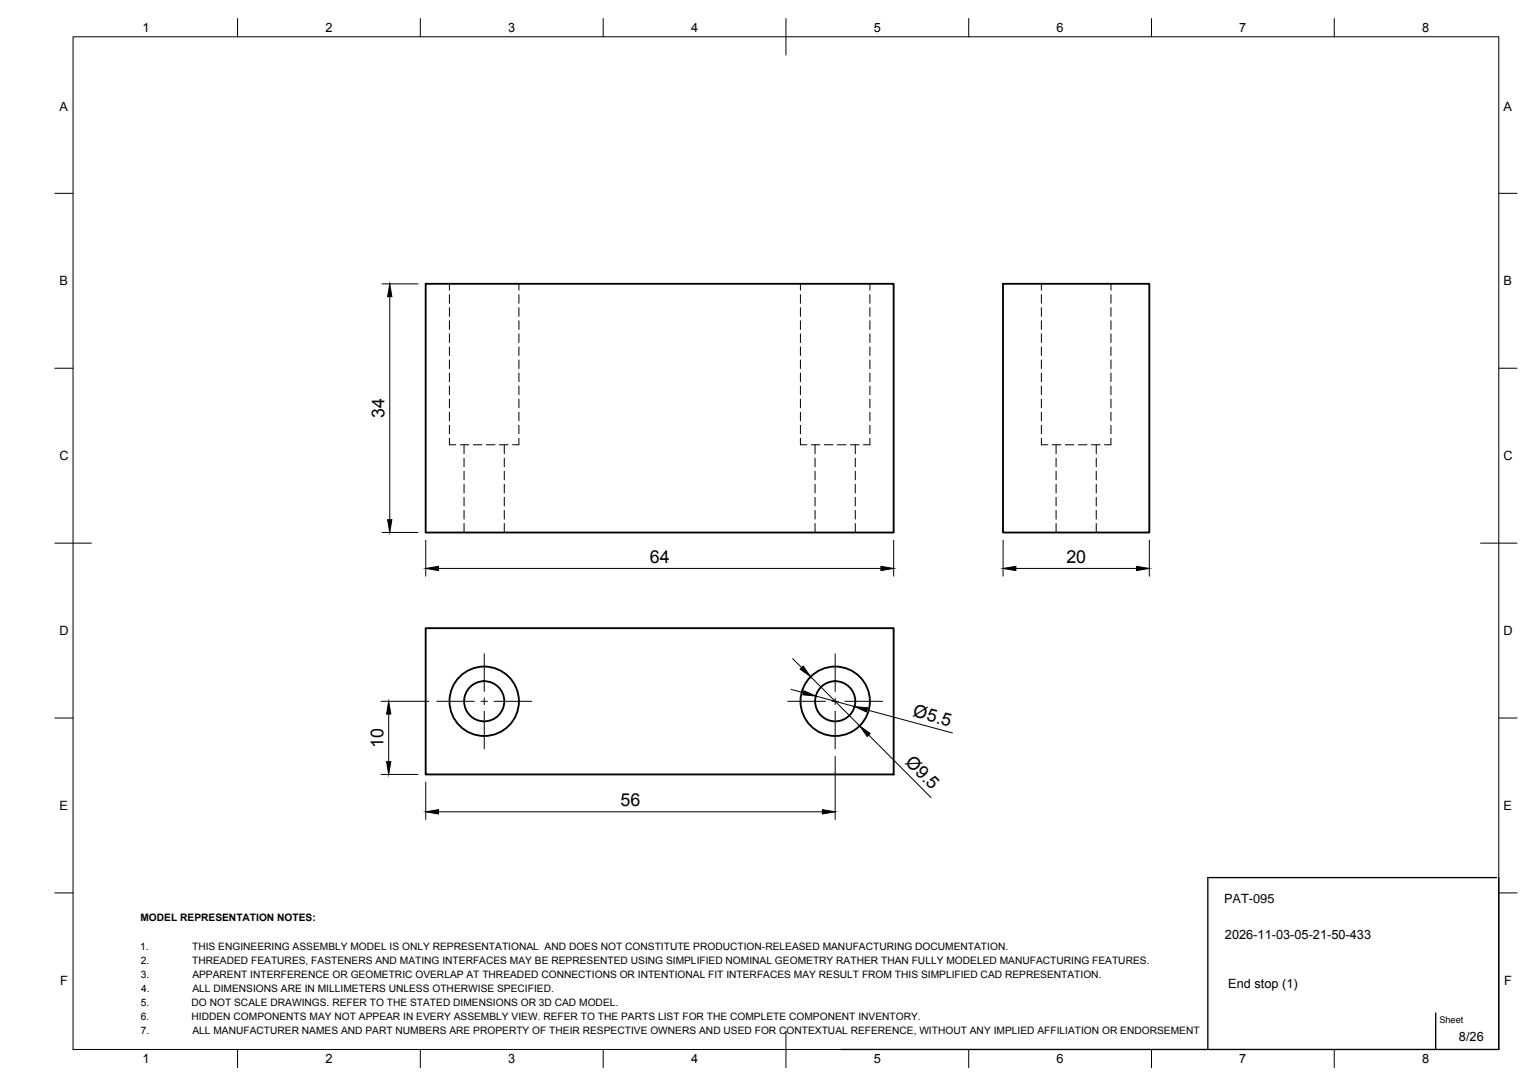
ISO-10303-21;
HEADER;
/* Generated by software containing ST-Developer
 * from STEP Tools, Inc. (www.steptools.com) 
 */

FILE_DESCRIPTION(
/* description */ ('Single-Axis Profile-Rail Linear Slide'),
/* implementation_level */ '2;1');

FILE_NAME(
/* name */ 'End stop (1).step',
/* time_stamp */ '2026-10-27T10:47:43-07:00',
/* author */ (''),
/* organization */ (''),
/* preprocessor_version */ 'ST-DEVELOPER v20.2',
/* originating_system */ 'Autodesk Translation Framework v15.17.0.0',
/* authorisation */ '');

FILE_SCHEMA (('AUTOMOTIVE_DESIGN { 1 0 10303 214 3 1 1 }'));
ENDSEC;

DATA;
#10=MECHANICAL_DESIGN_GEOMETRIC_PRESENTATION_REPRESENTATION('',(#332),#14478);
#278=SHAPE_REPRESENTATION_RELATIONSHIP('SRR','None',#14608,#305);
#305=ADVANCED_BREP_SHAPE_REPRESENTATION('',(#359),#14452);
#332=STYLED_ITEM('',(#14824),#359);
#359=MANIFOLD_SOLID_BREP('Body1',#8592);
#412=FACE_BOUND('',#1369,.T.);
#413=FACE_BOUND('',#1372,.T.);
#414=FACE_BOUND('',#1380,.T.);
#415=FACE_BOUND('',#1381,.T.);
#416=FACE_BOUND('',#1383,.T.);
#417=FACE_BOUND('',#1384,.T.);
#488=PLANE('',#9002);
#489=PLANE('',#9007);
#490=PLANE('',#9013);
#491=PLANE('',#9014);
#492=PLANE('',#9015);
#493=PLANE('',#9016);
#494=PLANE('',#9017);
#495=PLANE('',#9018);
#878=FACE_OUTER_BOUND('',#1367,.T.);
#879=FACE_OUTER_BOUND('',#1368,.T.);
#880=FACE_OUTER_BOUND('',#1370,.T.);
#881=FACE_OUTER_BOUND('',#1371,.T.);
#882=FACE_OUTER_BOUND('',#1373,.T.);
#883=FACE_OUTER_BOUND('',#1374,.T.);
#884=FACE_OUTER_BOUND('',#1375,.T.);
#885=FACE_OUTER_BOUND('',#1376,.T.);
#886=FACE_OUTER_BOUND('',#1377,.T.);
#887=FACE_OUTER_BOUND('',#1378,.T.);
#888=FACE_OUTER_BOUND('',#1379,.T.);
#889=FACE_OUTER_BOUND('',#1382,.T.);
#1367=EDGE_LOOP('',(#5993,#5994,#5995,#5996));
#1368=EDGE_LOOP('',(#5997));
#1369=EDGE_LOOP('',(#5998));
#1370=EDGE_LOOP('',(#5999,#6000,#6001,#6002));
#1371=EDGE_LOOP('',(#6003));
#1372=EDGE_LOOP('',(#6004));
#1373=EDGE_LOOP('',(#6005,#6006,#6007,#6008));
#1374=EDGE_LOOP('',(#6009,#6010,#6011,#6012));
#1375=EDGE_LOOP('',(#6013,#6014,#6015,#6016));
#1376=EDGE_LOOP('',(#6017,#6018,#6019,#6020));
#1377=EDGE_LOOP('',(#6021,#6022,#6023,#6024));
#1378=EDGE_LOOP('',(#6025,#6026,#6027,#6028));
#1379=EDGE_LOOP('',(#6029,#6030,#6031,#6032));
#1380=EDGE_LOOP('',(#6033));
#1381=EDGE_LOOP('',(#6034));
#1382=EDGE_LOOP('',(#6035,#6036,#6037,#6038));
#1383=EDGE_LOOP('',(#6039));
#1384=EDGE_LOOP('',(#6040));
#1894=LINE('',#12194,#2865);
#1895=LINE('',#12203,#2866);
#1896=LINE('',#12211,#2867);
#1897=LINE('',#12215,#2868);
#1898=LINE('',#12219,#2869);
#1899=LINE('',#12221,#2870);
#1900=LINE('',#12223,#2871);
#1901=LINE('',#12224,#2872);
#1902=LINE('',#12227,#2873);
#1903=LINE('',#12229,#2874);
#1904=LINE('',#12230,#2875);
#1905=LINE('',#12233,#2876);
#1906=LINE('',#12235,#2877);
#1907=LINE('',#12236,#2878);
#1908=LINE('',#12238,#2879);
#1909=LINE('',#12239,#2880);
#2865=VECTOR('',#9839,0.475000000000001);
#2866=VECTOR('',#9850,0.475000000000001);
#2867=VECTOR('',#9861,0.274999999999999);
#2868=VECTOR('',#9866,0.274999999999999);
#2869=VECTOR('',#9869,1.);
#2870=VECTOR('',#9870,1.);
#2871=VECTOR('',#9871,1.);
#2872=VECTOR('',#9872,1.);
#2873=VECTOR('',#9875,1.);
#2874=VECTOR('',#9876,1.);
#2875=VECTOR('',#9877,1.);
#2876=VECTOR('',#9880,1.);
#2877=VECTOR('',#9881,1.);
#2878=VECTOR('',#9882,1.);
#2879=VECTOR('',#9885,1.);
#2880=VECTOR('',#9886,1.);
#3818=CIRCLE('',#9000,0.475000000000001);
#3819=CIRCLE('',#9001,0.475000000000001);
#3820=CIRCLE('',#9003,0.274999999999999);
#3821=CIRCLE('',#9005,0.475000000000001);
#3822=CIRCLE('',#9006,0.475000000000001);
#3823=CIRCLE('',#9008,0.274999999999999);
#3824=CIRCLE('',#9010,0.274999999999999);
#3825=CIRCLE('',#9012,0.274999999999999);
#3998=VERTEX_POINT('',#12191);
#3999=VERTEX_POINT('',#12193);
#4000=VERTEX_POINT('',#12197);
#4001=VERTEX_POINT('',#12200);
#4002=VERTEX_POINT('',#12202);
#4003=VERTEX_POINT('',#12206);
#4004=VERTEX_POINT('',#12209);
#4005=VERTEX_POINT('',#12213);
#4006=VERTEX_POINT('',#12217);
#4007=VERTEX_POINT('',#12218);
#4008=VERTEX_POINT('',#12220);
#4009=VERTEX_POINT('',#12222);
#4010=VERTEX_POINT('',#12226);
#4011=VERTEX_POINT('',#12228);
#4012=VERTEX_POINT('',#12232);
#4013=VERTEX_POINT('',#12234);
#4774=EDGE_CURVE('',#3998,#3998,#3818,.T.);
#4775=EDGE_CURVE('',#3998,#3999,#1894,.T.);
#4776=EDGE_CURVE('',#3999,#3999,#3819,.T.);
#4777=EDGE_CURVE('',#4000,#4000,#3820,.T.);
#4778=EDGE_CURVE('',#4001,#4001,#3821,.T.);
#4779=EDGE_CURVE('',#4001,#4002,#1895,.T.);
#4780=EDGE_CURVE('',#4002,#4002,#3822,.T.);
#4781=EDGE_CURVE('',#4003,#4003,#3823,.T.);
#4782=EDGE_CURVE('',#4004,#4004,#3824,.T.);
#4783=EDGE_CURVE('',#4004,#4000,#1896,.T.);
#4784=EDGE_CURVE('',#4005,#4005,#3825,.T.);
#4785=EDGE_CURVE('',#4005,#4003,#1897,.T.);
#4786=EDGE_CURVE('',#4006,#4007,#1898,.T.);
#4787=EDGE_CURVE('',#4007,#4008,#1899,.T.);
#4788=EDGE_CURVE('',#4009,#4008,#1900,.T.);
#4789=EDGE_CURVE('',#4006,#4009,#1901,.T.);
#4790=EDGE_CURVE('',#4010,#4006,#1902,.T.);
#4791=EDGE_CURVE('',#4011,#4009,#1903,.T.);
#4792=EDGE_CURVE('',#4010,#4011,#1904,.T.);
#4793=EDGE_CURVE('',#4012,#4010,#1905,.T.);
#4794=EDGE_CURVE('',#4013,#4011,#1906,.T.);
#4795=EDGE_CURVE('',#4012,#4013,#1907,.T.);
#4796=EDGE_CURVE('',#4007,#4012,#1908,.T.);
#4797=EDGE_CURVE('',#4008,#4013,#1909,.T.);
#5993=ORIENTED_EDGE('',*,*,#4774,.F.);
#5994=ORIENTED_EDGE('',*,*,#4775,.T.);
#5995=ORIENTED_EDGE('',*,*,#4776,.F.);
#5996=ORIENTED_EDGE('',*,*,#4775,.F.);
#5997=ORIENTED_EDGE('',*,*,#4774,.T.);
#5998=ORIENTED_EDGE('',*,*,#4777,.F.);
#5999=ORIENTED_EDGE('',*,*,#4778,.F.);
#6000=ORIENTED_EDGE('',*,*,#4779,.T.);
#6001=ORIENTED_EDGE('',*,*,#4780,.F.);
#6002=ORIENTED_EDGE('',*,*,#4779,.F.);
#6003=ORIENTED_EDGE('',*,*,#4778,.T.);
#6004=ORIENTED_EDGE('',*,*,#4781,.F.);
#6005=ORIENTED_EDGE('',*,*,#4782,.F.);
#6006=ORIENTED_EDGE('',*,*,#4783,.T.);
#6007=ORIENTED_EDGE('',*,*,#4777,.T.);
#6008=ORIENTED_EDGE('',*,*,#4783,.F.);
#6009=ORIENTED_EDGE('',*,*,#4784,.F.);
#6010=ORIENTED_EDGE('',*,*,#4785,.T.);
#6011=ORIENTED_EDGE('',*,*,#4781,.T.);
#6012=ORIENTED_EDGE('',*,*,#4785,.F.);
#6013=ORIENTED_EDGE('',*,*,#4786,.T.);
#6014=ORIENTED_EDGE('',*,*,#4787,.T.);
#6015=ORIENTED_EDGE('',*,*,#4788,.F.);
#6016=ORIENTED_EDGE('',*,*,#4789,.F.);
#6017=ORIENTED_EDGE('',*,*,#4790,.T.);
#6018=ORIENTED_EDGE('',*,*,#4789,.T.);
#6019=ORIENTED_EDGE('',*,*,#4791,.F.);
#6020=ORIENTED_EDGE('',*,*,#4792,.F.);
#6021=ORIENTED_EDGE('',*,*,#4793,.T.);
#6022=ORIENTED_EDGE('',*,*,#4792,.T.);
#6023=ORIENTED_EDGE('',*,*,#4794,.F.);
#6024=ORIENTED_EDGE('',*,*,#4795,.F.);
#6025=ORIENTED_EDGE('',*,*,#4796,.T.);
#6026=ORIENTED_EDGE('',*,*,#4795,.T.);
#6027=ORIENTED_EDGE('',*,*,#4797,.F.);
#6028=ORIENTED_EDGE('',*,*,#4787,.F.);
#6029=ORIENTED_EDGE('',*,*,#4797,.T.);
#6030=ORIENTED_EDGE('',*,*,#4794,.T.);
#6031=ORIENTED_EDGE('',*,*,#4791,.T.);
#6032=ORIENTED_EDGE('',*,*,#4788,.T.);
#6033=ORIENTED_EDGE('',*,*,#4776,.T.);
#6034=ORIENTED_EDGE('',*,*,#4780,.T.);
#6035=ORIENTED_EDGE('',*,*,#4796,.F.);
#6036=ORIENTED_EDGE('',*,*,#4786,.F.);
#6037=ORIENTED_EDGE('',*,*,#4790,.F.);
#6038=ORIENTED_EDGE('',*,*,#4793,.F.);
#6039=ORIENTED_EDGE('',*,*,#4782,.T.);
#6040=ORIENTED_EDGE('',*,*,#4784,.T.);
#8089=CYLINDRICAL_SURFACE('',#8999,0.475000000000001);
#8090=CYLINDRICAL_SURFACE('',#9004,0.475000000000001);
#8091=CYLINDRICAL_SURFACE('',#9009,0.274999999999999);
#8092=CYLINDRICAL_SURFACE('',#9011,0.274999999999999);
#8172=ADVANCED_FACE('',(#878),#8089,.F.);
#8173=ADVANCED_FACE('',(#879,#412),#488,.T.);
#8174=ADVANCED_FACE('',(#880),#8090,.F.);
#8175=ADVANCED_FACE('',(#881,#413),#489,.T.);
#8176=ADVANCED_FACE('',(#882),#8091,.F.);
#8177=ADVANCED_FACE('',(#883),#8092,.F.);
#8178=ADVANCED_FACE('',(#884),#490,.T.);
#8179=ADVANCED_FACE('',(#885),#491,.T.);
#8180=ADVANCED_FACE('',(#886),#492,.T.);
#8181=ADVANCED_FACE('',(#887),#493,.T.);
#8182=ADVANCED_FACE('',(#888,#414,#415),#494,.T.);
#8183=ADVANCED_FACE('',(#889,#416,#417),#495,.F.);
#8592=CLOSED_SHELL('',(#8172,#8173,#8174,#8175,#8176,#8177,#8178,#8179,
#8180,#8181,#8182,#8183));
#8998=AXIS2_PLACEMENT_3D('',#12189,#9833,#9834);
#8999=AXIS2_PLACEMENT_3D('',#12190,#9835,#9836);
#9000=AXIS2_PLACEMENT_3D('',#12192,#9837,#9838);
#9001=AXIS2_PLACEMENT_3D('',#12195,#9840,#9841);
#9002=AXIS2_PLACEMENT_3D('',#12196,#9842,#9843);
#9003=AXIS2_PLACEMENT_3D('',#12198,#9844,#9845);
#9004=AXIS2_PLACEMENT_3D('',#12199,#9846,#9847);
#9005=AXIS2_PLACEMENT_3D('',#12201,#9848,#9849);
#9006=AXIS2_PLACEMENT_3D('',#12204,#9851,#9852);
#9007=AXIS2_PLACEMENT_3D('',#12205,#9853,#9854);
#9008=AXIS2_PLACEMENT_3D('',#12207,#9855,#9856);
#9009=AXIS2_PLACEMENT_3D('',#12208,#9857,#9858);
#9010=AXIS2_PLACEMENT_3D('',#12210,#9859,#9860);
#9011=AXIS2_PLACEMENT_3D('',#12212,#9862,#9863);
#9012=AXIS2_PLACEMENT_3D('',#12214,#9864,#9865);
#9013=AXIS2_PLACEMENT_3D('',#12216,#9867,#9868);
#9014=AXIS2_PLACEMENT_3D('',#12225,#9873,#9874);
#9015=AXIS2_PLACEMENT_3D('',#12231,#9878,#9879);
#9016=AXIS2_PLACEMENT_3D('',#12237,#9883,#9884);
#9017=AXIS2_PLACEMENT_3D('',#12240,#9887,#9888);
#9018=AXIS2_PLACEMENT_3D('',#12241,#9889,#9890);
#9833=DIRECTION('axis',(0.,0.,1.));
#9834=DIRECTION('refdir',(1.,0.,0.));
#9835=DIRECTION('center_axis',(0.,0.,1.));
#9836=DIRECTION('ref_axis',(1.,0.,0.));
#9837=DIRECTION('center_axis',(0.,0.,1.));
#9838=DIRECTION('ref_axis',(1.,0.,0.));
#9839=DIRECTION('',(0.,0.,1.));
#9840=DIRECTION('center_axis',(0.,0.,-1.));
#9841=DIRECTION('ref_axis',(1.,0.,0.));
#9842=DIRECTION('center_axis',(0.,0.,1.));
#9843=DIRECTION('ref_axis',(1.,0.,0.));
#9844=DIRECTION('center_axis',(0.,0.,1.));
#9845=DIRECTION('ref_axis',(1.,0.,0.));
#9846=DIRECTION('center_axis',(0.,0.,1.));
#9847=DIRECTION('ref_axis',(1.,0.,0.));
#9848=DIRECTION('center_axis',(0.,0.,1.));
#9849=DIRECTION('ref_axis',(1.,0.,0.));
#9850=DIRECTION('',(0.,0.,1.));
#9851=DIRECTION('center_axis',(0.,0.,-1.));
#9852=DIRECTION('ref_axis',(1.,0.,0.));
#9853=DIRECTION('center_axis',(0.,0.,1.));
#9854=DIRECTION('ref_axis',(1.,0.,0.));
#9855=DIRECTION('center_axis',(0.,0.,1.));
#9856=DIRECTION('ref_axis',(1.,0.,0.));
#9857=DIRECTION('center_axis',(0.,0.,1.));
#9858=DIRECTION('ref_axis',(1.,0.,0.));
#9859=DIRECTION('center_axis',(0.,0.,1.));
#9860=DIRECTION('ref_axis',(1.,0.,0.));
#9861=DIRECTION('',(0.,0.,1.));
#9862=DIRECTION('center_axis',(0.,0.,1.));
#9863=DIRECTION('ref_axis',(1.,0.,0.));
#9864=DIRECTION('center_axis',(0.,0.,1.));
#9865=DIRECTION('ref_axis',(1.,0.,0.));
#9866=DIRECTION('',(0.,0.,1.));
#9867=DIRECTION('center_axis',(0.,1.,0.));
#9868=DIRECTION('ref_axis',(-1.,0.,0.));
#9869=DIRECTION('',(-1.,0.,0.));
#9870=DIRECTION('',(0.,0.,1.));
#9871=DIRECTION('',(-1.,0.,0.));
#9872=DIRECTION('',(0.,0.,1.));
#9873=DIRECTION('center_axis',(1.,0.,0.));
#9874=DIRECTION('ref_axis',(0.,1.,0.));
#9875=DIRECTION('',(0.,1.,0.));
#9876=DIRECTION('',(0.,1.,0.));
#9877=DIRECTION('',(0.,0.,1.));
#9878=DIRECTION('center_axis',(0.,-1.,0.));
#9879=DIRECTION('ref_axis',(1.,0.,0.));
#9880=DIRECTION('',(1.,0.,0.));
#9881=DIRECTION('',(1.,0.,0.));
#9882=DIRECTION('',(0.,0.,1.));
#9883=DIRECTION('center_axis',(-1.,0.,0.));
#9884=DIRECTION('ref_axis',(0.,-1.,0.));
#9885=DIRECTION('',(0.,-1.,0.));
#9886=DIRECTION('',(0.,-1.,0.));
#9887=DIRECTION('center_axis',(0.,0.,1.));
#9888=DIRECTION('ref_axis',(1.,0.,0.));
#9889=DIRECTION('center_axis',(0.,0.,1.));
#9890=DIRECTION('ref_axis',(1.,0.,0.));
#12189=CARTESIAN_POINT('',(0.,0.,0.));
#12190=CARTESIAN_POINT('Origin',(23.,-2.4,4.));
#12191=CARTESIAN_POINT('',(22.525,-2.4,4.));
#12192=CARTESIAN_POINT('Origin',(23.,-2.4,4.));
#12193=CARTESIAN_POINT('',(22.525,-2.4,6.2));
#12194=CARTESIAN_POINT('',(22.525,-2.4,4.));
#12195=CARTESIAN_POINT('Origin',(23.,-2.4,6.2));
#12196=CARTESIAN_POINT('Origin',(23.,-2.4,4.));
#12197=CARTESIAN_POINT('',(22.725,-2.4,4.));
#12198=CARTESIAN_POINT('Origin',(23.,-2.4,4.));
#12199=CARTESIAN_POINT('Origin',(23.,2.4,4.));
#12200=CARTESIAN_POINT('',(22.525,2.4,4.));
#12201=CARTESIAN_POINT('Origin',(23.,2.4,4.));
#12202=CARTESIAN_POINT('',(22.525,2.4,6.2));
#12203=CARTESIAN_POINT('',(22.525,2.4,4.));
#12204=CARTESIAN_POINT('Origin',(23.,2.4,6.2));
#12205=CARTESIAN_POINT('Origin',(23.,2.4,4.));
#12206=CARTESIAN_POINT('',(22.725,2.4,4.));
#12207=CARTESIAN_POINT('Origin',(23.,2.4,4.));
#12208=CARTESIAN_POINT('Origin',(23.,-2.4,2.7));
#12209=CARTESIAN_POINT('',(22.725,-2.4,2.8));
#12210=CARTESIAN_POINT('Origin',(23.,-2.4,2.8));
#12211=CARTESIAN_POINT('',(22.725,-2.4,2.7));
#12212=CARTESIAN_POINT('Origin',(23.,2.4,2.7));
#12213=CARTESIAN_POINT('',(22.725,2.4,2.8));
#12214=CARTESIAN_POINT('Origin',(23.,2.4,2.8));
#12215=CARTESIAN_POINT('',(22.725,2.4,2.7));
#12216=CARTESIAN_POINT('Origin',(24.,3.2,2.8));
#12217=CARTESIAN_POINT('',(24.,3.2,2.8));
#12218=CARTESIAN_POINT('',(22.,3.2,2.8));
#12219=CARTESIAN_POINT('',(24.,3.2,2.8));
#12220=CARTESIAN_POINT('',(22.,3.2,6.2));
#12221=CARTESIAN_POINT('',(22.,3.2,2.8));
#12222=CARTESIAN_POINT('',(24.,3.2,6.2));
#12223=CARTESIAN_POINT('',(24.,3.2,6.2));
#12224=CARTESIAN_POINT('',(24.,3.2,2.8));
#12225=CARTESIAN_POINT('Origin',(24.,-3.2,2.8));
#12226=CARTESIAN_POINT('',(24.,-3.2,2.8));
#12227=CARTESIAN_POINT('',(24.,-3.2,2.8));
#12228=CARTESIAN_POINT('',(24.,-3.2,6.2));
#12229=CARTESIAN_POINT('',(24.,-3.2,6.2));
#12230=CARTESIAN_POINT('',(24.,-3.2,2.8));
#12231=CARTESIAN_POINT('Origin',(22.,-3.2,2.8));
#12232=CARTESIAN_POINT('',(22.,-3.2,2.8));
#12233=CARTESIAN_POINT('',(22.,-3.2,2.8));
#12234=CARTESIAN_POINT('',(22.,-3.2,6.2));
#12235=CARTESIAN_POINT('',(22.,-3.2,6.2));
#12236=CARTESIAN_POINT('',(22.,-3.2,2.8));
#12237=CARTESIAN_POINT('Origin',(22.,3.2,2.8));
#12238=CARTESIAN_POINT('',(22.,3.2,2.8));
#12239=CARTESIAN_POINT('',(22.,3.2,6.2));
#12240=CARTESIAN_POINT('Origin',(23.,0.,6.2));
#12241=CARTESIAN_POINT('Origin',(23.,0.,2.8));
#14420=UNCERTAINTY_MEASURE_WITH_UNIT(LENGTH_MEASURE(0.001),#14479,
'DISTANCE_ACCURACY_VALUE',
'Maximum model space distance between geometric entities at asserted c
onnectivities');
#14446=UNCERTAINTY_MEASURE_WITH_UNIT(LENGTH_MEASURE(0.001),#14479,
'DISTANCE_ACCURACY_VALUE',
'Maximum model space distance between geometric entities at asserted c
onnectivities');
#14452=(
GEOMETRIC_REPRESENTATION_CONTEXT(3)
GLOBAL_UNCERTAINTY_ASSIGNED_CONTEXT((#14420))
GLOBAL_UNIT_ASSIGNED_CONTEXT((#14479,#14481,#14482))
REPRESENTATION_CONTEXT('','3D')
);
#14478=(
GEOMETRIC_REPRESENTATION_CONTEXT(3)
GLOBAL_UNCERTAINTY_ASSIGNED_CONTEXT((#14446))
GLOBAL_UNIT_ASSIGNED_CONTEXT((#14479,#14481,#14482))
REPRESENTATION_CONTEXT('','3D')
);
#14479=(
LENGTH_UNIT()
NAMED_UNIT(*)
SI_UNIT(.CENTI.,.METRE.)
);
#14481=(
NAMED_UNIT(*)
PLANE_ANGLE_UNIT()
SI_UNIT($,.RADIAN.)
);
#14482=(
NAMED_UNIT(*)
SI_UNIT($,.STERADIAN.)
SOLID_ANGLE_UNIT()
);
#14488=SHAPE_DEFINITION_REPRESENTATION(#14519,#14608);
#14519=PRODUCT_DEFINITION_SHAPE('',$,#14640);
#14608=SHAPE_REPRESENTATION('',(#8998),#14452);
#14634=PRODUCT_DEFINITION_CONTEXT('part definition',#14729,'design');
#14640=PRODUCT_DEFINITION('End stop (1)','End stop (1)',#14671,#14634);
#14671=PRODUCT_DEFINITION_FORMATION('',$,#14736);
#14729=APPLICATION_CONTEXT(
'Core Data for Automotive Mechanical Design Process');
#14730=PRODUCT_CONTEXT('part definition',#14729,'mechanical');
#14736=PRODUCT('End stop (1)','End stop (1)','End stop (1)',(#14730));
#14818=COLOUR_RGB('Sky Blue',0.24,0.69,0.87);
#14819=FILL_AREA_STYLE_COLOUR('',#14818);
#14820=FILL_AREA_STYLE('',(#14819));
#14821=SURFACE_STYLE_FILL_AREA(#14820);
#14822=SURFACE_SIDE_STYLE('',(#14821));
#14823=SURFACE_STYLE_USAGE(.BOTH.,#14822);
#14824=PRESENTATION_STYLE_ASSIGNMENT((#14823));
ENDSEC;
END-ISO-10303-21;
